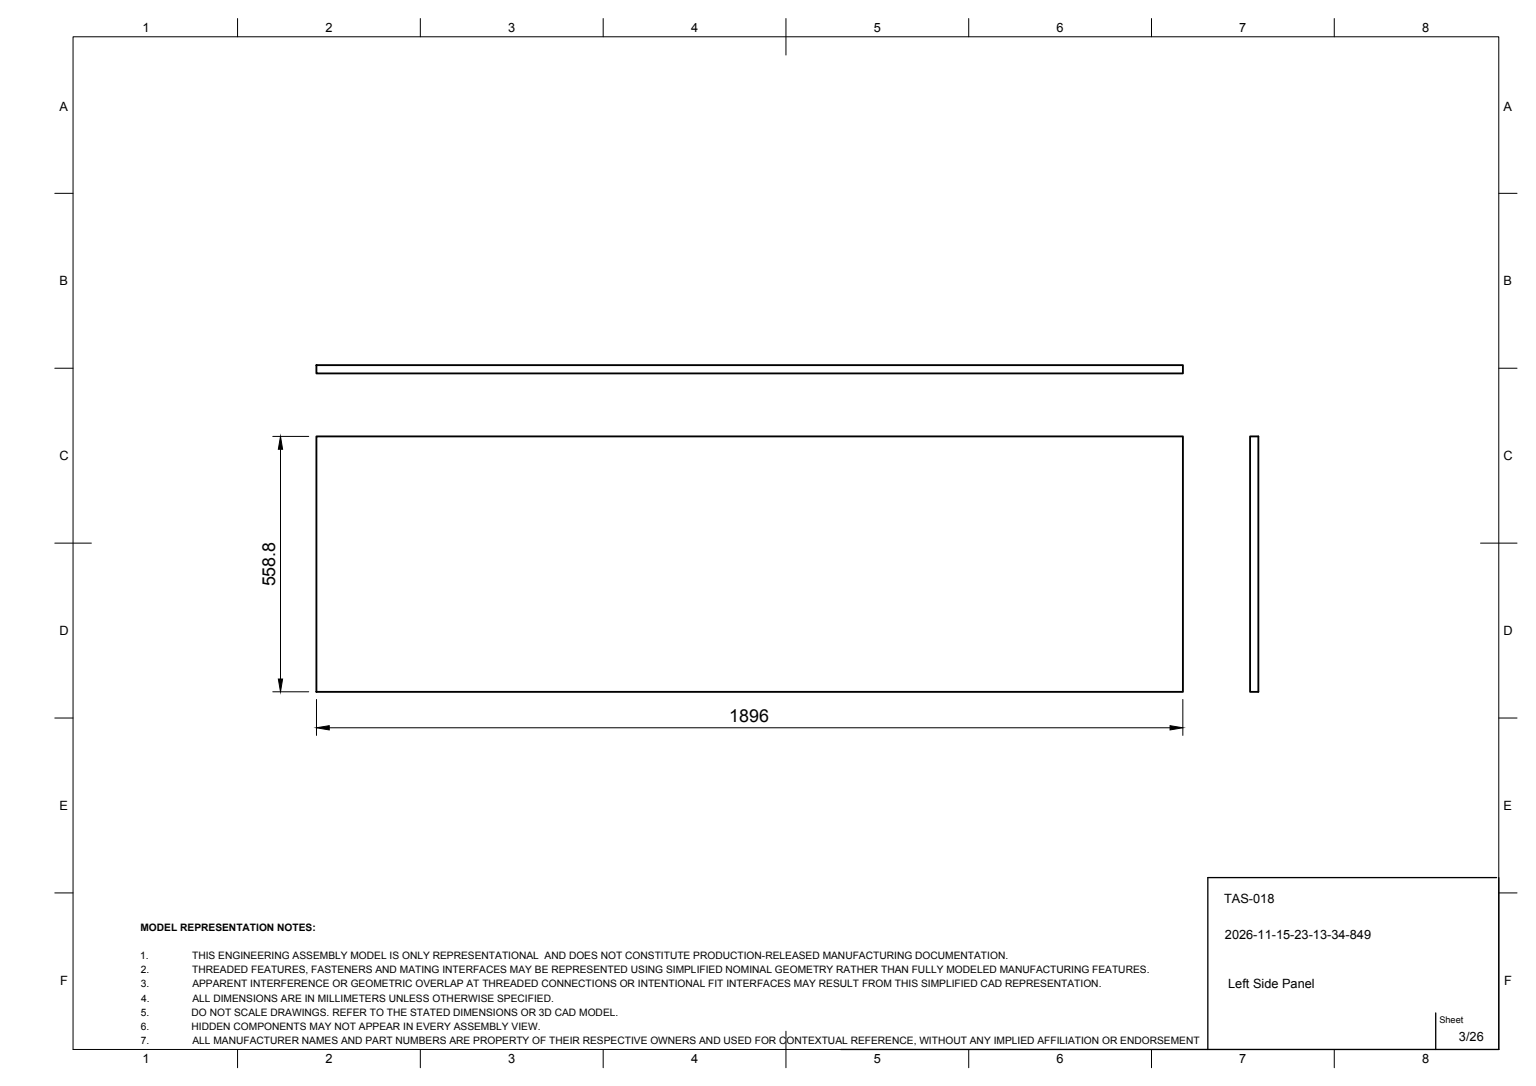
ISO-10303-21;
HEADER;
/* Generated by software containing ST-Developer
 * from STEP Tools, Inc. (www.steptools.com) 
 */

FILE_DESCRIPTION(
/* description */ (''),
/* implementation_level */ '2;1');

FILE_NAME(
/* name */ 'Left Side Panel.step',
/* time_stamp */ '2026-11-15T15:17:57-08:00',
/* author */ (''),
/* organization */ (''),
/* preprocessor_version */ 'ST-DEVELOPER v20.2',
/* originating_system */ 'Autodesk Translation Framework v15.17.0.0',
/* authorisation */ '');

FILE_SCHEMA (('AUTOMOTIVE_DESIGN { 1 0 10303 214 3 1 1 }'));
ENDSEC;

DATA;
#10=MECHANICAL_DESIGN_GEOMETRIC_PRESENTATION_REPRESENTATION('',(#178),#3723);
#130=SHAPE_REPRESENTATION_RELATIONSHIP('SRR','None',#3811,#154);
#154=ADVANCED_BREP_SHAPE_REPRESENTATION('',(#202),#3700);
#178=STYLED_ITEM('',(#3943),#202);
#202=MANIFOLD_SOLID_BREP('Body1',#2026);
#231=FACE_OUTER_BOUND('',#357,.T.);
#232=FACE_OUTER_BOUND('',#358,.T.);
#233=FACE_OUTER_BOUND('',#359,.T.);
#234=FACE_OUTER_BOUND('',#360,.T.);
#235=FACE_OUTER_BOUND('',#361,.T.);
#236=FACE_OUTER_BOUND('',#362,.T.);
#357=EDGE_LOOP('',(#1335,#1336,#1337,#1338));
#358=EDGE_LOOP('',(#1339,#1340,#1341,#1342));
#359=EDGE_LOOP('',(#1343,#1344,#1345,#1346));
#360=EDGE_LOOP('',(#1347,#1348,#1349,#1350));
#361=EDGE_LOOP('',(#1351,#1352,#1353,#1354));
#362=EDGE_LOOP('',(#1355,#1356,#1357,#1358));
#489=LINE('',#3137,#711);
#490=LINE('',#3139,#712);
#491=LINE('',#3141,#713);
#492=LINE('',#3142,#714);
#493=LINE('',#3145,#715);
#494=LINE('',#3147,#716);
#495=LINE('',#3148,#717);
#496=LINE('',#3151,#718);
#497=LINE('',#3153,#719);
#498=LINE('',#3154,#720);
#499=LINE('',#3156,#721);
#500=LINE('',#3157,#722);
#711=VECTOR('',#2539,74.6456692913386);
#712=VECTOR('',#2540,22.);
#713=VECTOR('',#2541,74.6456692913386);
#714=VECTOR('',#2542,22.);
#715=VECTOR('',#2545,0.708661417322833);
#716=VECTOR('',#2546,22.);
#717=VECTOR('',#2547,0.708661417322833);
#718=VECTOR('',#2550,74.6456692913386);
#719=VECTOR('',#2551,22.);
#720=VECTOR('',#2552,74.6456692913386);
#721=VECTOR('',#2555,0.708661417322833);
#722=VECTOR('',#2556,0.708661417322833);
#929=VERTEX_POINT('',#3135);
#930=VERTEX_POINT('',#3136);
#931=VERTEX_POINT('',#3138);
#932=VERTEX_POINT('',#3140);
#933=VERTEX_POINT('',#3144);
#934=VERTEX_POINT('',#3146);
#935=VERTEX_POINT('',#3150);
#936=VERTEX_POINT('',#3152);
#1089=EDGE_CURVE('',#929,#930,#489,.T.);
#1090=EDGE_CURVE('',#931,#930,#490,.T.);
#1091=EDGE_CURVE('',#932,#931,#491,.T.);
#1092=EDGE_CURVE('',#932,#929,#492,.T.);
#1093=EDGE_CURVE('',#930,#933,#493,.T.);
#1094=EDGE_CURVE('',#934,#933,#494,.T.);
#1095=EDGE_CURVE('',#931,#934,#495,.T.);
#1096=EDGE_CURVE('',#933,#935,#496,.T.);
#1097=EDGE_CURVE('',#936,#935,#497,.T.);
#1098=EDGE_CURVE('',#934,#936,#498,.T.);
#1099=EDGE_CURVE('',#935,#929,#499,.T.);
#1100=EDGE_CURVE('',#936,#932,#500,.T.);
#1335=ORIENTED_EDGE('',*,*,#1089,.T.);
#1336=ORIENTED_EDGE('',*,*,#1090,.F.);
#1337=ORIENTED_EDGE('',*,*,#1091,.F.);
#1338=ORIENTED_EDGE('',*,*,#1092,.T.);
#1339=ORIENTED_EDGE('',*,*,#1093,.T.);
#1340=ORIENTED_EDGE('',*,*,#1094,.F.);
#1341=ORIENTED_EDGE('',*,*,#1095,.F.);
#1342=ORIENTED_EDGE('',*,*,#1090,.T.);
#1343=ORIENTED_EDGE('',*,*,#1096,.T.);
#1344=ORIENTED_EDGE('',*,*,#1097,.F.);
#1345=ORIENTED_EDGE('',*,*,#1098,.F.);
#1346=ORIENTED_EDGE('',*,*,#1094,.T.);
#1347=ORIENTED_EDGE('',*,*,#1099,.T.);
#1348=ORIENTED_EDGE('',*,*,#1092,.F.);
#1349=ORIENTED_EDGE('',*,*,#1100,.F.);
#1350=ORIENTED_EDGE('',*,*,#1097,.T.);
#1351=ORIENTED_EDGE('',*,*,#1091,.T.);
#1352=ORIENTED_EDGE('',*,*,#1095,.T.);
#1353=ORIENTED_EDGE('',*,*,#1098,.T.);
#1354=ORIENTED_EDGE('',*,*,#1100,.T.);
#1355=ORIENTED_EDGE('',*,*,#1089,.F.);
#1356=ORIENTED_EDGE('',*,*,#1099,.F.);
#1357=ORIENTED_EDGE('',*,*,#1096,.F.);
#1358=ORIENTED_EDGE('',*,*,#1093,.F.);
#1785=PLANE('',#2325);
#1786=PLANE('',#2326);
#1787=PLANE('',#2327);
#1788=PLANE('',#2328);
#1789=PLANE('',#2329);
#1790=PLANE('',#2330);
#1905=ADVANCED_FACE('',(#231),#1785,.F.);
#1906=ADVANCED_FACE('',(#232),#1786,.F.);
#1907=ADVANCED_FACE('',(#233),#1787,.F.);
#1908=ADVANCED_FACE('',(#234),#1788,.F.);
#1909=ADVANCED_FACE('',(#235),#1789,.T.);
#1910=ADVANCED_FACE('',(#236),#1790,.F.);
#2026=CLOSED_SHELL('',(#1905,#1906,#1907,#1908,#1909,#1910));
#2324=AXIS2_PLACEMENT_3D('',#3133,#2535,#2536);
#2325=AXIS2_PLACEMENT_3D('',#3134,#2537,#2538);
#2326=AXIS2_PLACEMENT_3D('',#3143,#2543,#2544);
#2327=AXIS2_PLACEMENT_3D('',#3149,#2548,#2549);
#2328=AXIS2_PLACEMENT_3D('',#3155,#2553,#2554);
#2329=AXIS2_PLACEMENT_3D('',#3158,#2557,#2558);
#2330=AXIS2_PLACEMENT_3D('',#3159,#2559,#2560);
#2535=DIRECTION('axis',(0.,0.,1.));
#2536=DIRECTION('refdir',(1.,0.,0.));
#2537=DIRECTION('center_axis',(1.,1.17112133399278E-16,0.));
#2538=DIRECTION('ref_axis',(0.,0.,-1.));
#2539=DIRECTION('',(1.49903530751076E-16,-1.,0.));
#2540=DIRECTION('',(0.,0.,-1.));
#2541=DIRECTION('',(1.49903530751076E-16,-1.,0.));
#2542=DIRECTION('',(0.,0.,-1.));
#2543=DIRECTION('center_axis',(0.,1.,0.));
#2544=DIRECTION('ref_axis',(0.,0.,1.));
#2545=DIRECTION('',(1.,0.,0.));
#2546=DIRECTION('',(0.,0.,-1.));
#2547=DIRECTION('',(1.,0.,0.));
#2548=DIRECTION('center_axis',(-1.,-1.17112133399278E-16,0.));
#2549=DIRECTION('ref_axis',(0.,0.,1.));
#2550=DIRECTION('',(-1.49903530751076E-16,1.,0.));
#2551=DIRECTION('',(0.,0.,-1.));
#2552=DIRECTION('',(-1.49903530751076E-16,1.,0.));
#2553=DIRECTION('center_axis',(0.,-1.,0.));
#2554=DIRECTION('ref_axis',(0.,0.,-1.));
#2555=DIRECTION('',(-1.,0.,0.));
#2556=DIRECTION('',(-1.,0.,0.));
#2557=DIRECTION('center_axis',(0.,0.,1.));
#2558=DIRECTION('ref_axis',(1.,0.,0.));
#2559=DIRECTION('center_axis',(0.,0.,1.));
#2560=DIRECTION('ref_axis',(1.,0.,0.));
#3133=CARTESIAN_POINT('',(0.,0.,0.));
#3134=CARTESIAN_POINT('Origin',(-36.,79.2913385826772,22.));
#3135=CARTESIAN_POINT('',(-36.,79.2913385826772,0.));
#3136=CARTESIAN_POINT('',(-36.,4.64566929133858,0.));
#3137=CARTESIAN_POINT('',(-36.,79.2913385826772,0.));
#3138=CARTESIAN_POINT('',(-36.,4.64566929133858,22.));
#3139=CARTESIAN_POINT('',(-36.,4.64566929133858,22.));
#3140=CARTESIAN_POINT('',(-36.,79.2913385826772,22.));
#3141=CARTESIAN_POINT('',(-36.,79.2913385826772,22.));
#3142=CARTESIAN_POINT('',(-36.,79.2913385826772,22.));
#3143=CARTESIAN_POINT('Origin',(-36.,4.64566929133858,22.));
#3144=CARTESIAN_POINT('',(-35.2913385826772,4.64566929133858,0.));
#3145=CARTESIAN_POINT('',(-36.,4.64566929133858,0.));
#3146=CARTESIAN_POINT('',(-35.2913385826772,4.64566929133858,22.));
#3147=CARTESIAN_POINT('',(-35.2913385826772,4.64566929133858,22.));
#3148=CARTESIAN_POINT('',(-36.,4.64566929133858,22.));
#3149=CARTESIAN_POINT('Origin',(-35.2913385826772,79.2913385826772,22.));
#3150=CARTESIAN_POINT('',(-35.2913385826772,79.2913385826772,0.));
#3151=CARTESIAN_POINT('',(-35.2913385826772,4.64566929133858,0.));
#3152=CARTESIAN_POINT('',(-35.2913385826772,79.2913385826772,22.));
#3153=CARTESIAN_POINT('',(-35.2913385826772,79.2913385826772,22.));
#3154=CARTESIAN_POINT('',(-35.2913385826772,4.64566929133858,22.));
#3155=CARTESIAN_POINT('Origin',(-36.,79.2913385826772,22.));
#3156=CARTESIAN_POINT('',(-35.2913385826772,79.2913385826772,0.));
#3157=CARTESIAN_POINT('',(-35.2913385826772,79.2913385826772,22.));
#3158=CARTESIAN_POINT('Origin',(0.,0.,22.));
#3159=CARTESIAN_POINT('Origin',(0.,0.,0.));
#3673=UNCERTAINTY_MEASURE_WITH_UNIT(LENGTH_MEASURE(0.000393700787401575),
#3725,'DISTANCE_ACCURACY_VALUE',
'Maximum model space distance between geometric entities at asserted c
onnectivities');
#3696=UNCERTAINTY_MEASURE_WITH_UNIT(LENGTH_MEASURE(0.000393700787401575),
#3725,'DISTANCE_ACCURACY_VALUE',
'Maximum model space distance between geometric entities at asserted c
onnectivities');
#3700=(
GEOMETRIC_REPRESENTATION_CONTEXT(3)
GLOBAL_UNCERTAINTY_ASSIGNED_CONTEXT((#3673))
GLOBAL_UNIT_ASSIGNED_CONTEXT((#3725,#3729,#3730))
REPRESENTATION_CONTEXT('','3D')
);
#3723=(
GEOMETRIC_REPRESENTATION_CONTEXT(3)
GLOBAL_UNCERTAINTY_ASSIGNED_CONTEXT((#3696))
GLOBAL_UNIT_ASSIGNED_CONTEXT((#3725,#3729,#3730))
REPRESENTATION_CONTEXT('','3D')
);
#3724=DIMENSIONAL_EXPONENTS(1.,0.,0.,0.,0.,0.,0.);
#3725=(
CONVERSION_BASED_UNIT('inch',#3728)
LENGTH_UNIT()
NAMED_UNIT(#3724)
);
#3726=(
LENGTH_UNIT()
NAMED_UNIT(*)
SI_UNIT(.MILLI.,.METRE.)
);
#3728=LENGTH_MEASURE_WITH_UNIT(LENGTH_MEASURE(25.4),#3726);
#3729=(
NAMED_UNIT(*)
PLANE_ANGLE_UNIT()
SI_UNIT($,.RADIAN.)
);
#3730=(
NAMED_UNIT(*)
SI_UNIT($,.STERADIAN.)
SOLID_ANGLE_UNIT()
);
#3734=SHAPE_DEFINITION_REPRESENTATION(#3761,#3811);
#3761=PRODUCT_DEFINITION_SHAPE('',$,#3838);
#3811=SHAPE_REPRESENTATION('',(#2324),#3700);
#3834=PRODUCT_DEFINITION_CONTEXT('part definition',#3914,'design');
#3838=PRODUCT_DEFINITION('2026-11-15-23-13-34-849','Left Side Panel',#3864,
#3834);
#3864=PRODUCT_DEFINITION_FORMATION('',$,#3919);
#3914=APPLICATION_CONTEXT(
'Core Data for Automotive Mechanical Design Process');
#3915=PRODUCT_CONTEXT('part definition',#3914,'mechanical');
#3919=PRODUCT('2026-11-15-23-13-34-849','Left Side Panel',$,(#3915));
#3943=PRESENTATION_STYLE_ASSIGNMENT((#3951));
#3951=SURFACE_STYLE_USAGE(.BOTH.,#3959);
#3959=SURFACE_SIDE_STYLE('',(#3967));
#3967=SURFACE_STYLE_FILL_AREA(#3975);
#3975=FILL_AREA_STYLE('Dark Blue',(#3983));
#3983=FILL_AREA_STYLE_COLOUR('Dark Blue',#3991);
#3991=COLOUR_RGB('Dark Blue',0.,0.125490196078431,0.376470588235294);
ENDSEC;
END-ISO-10303-21;
